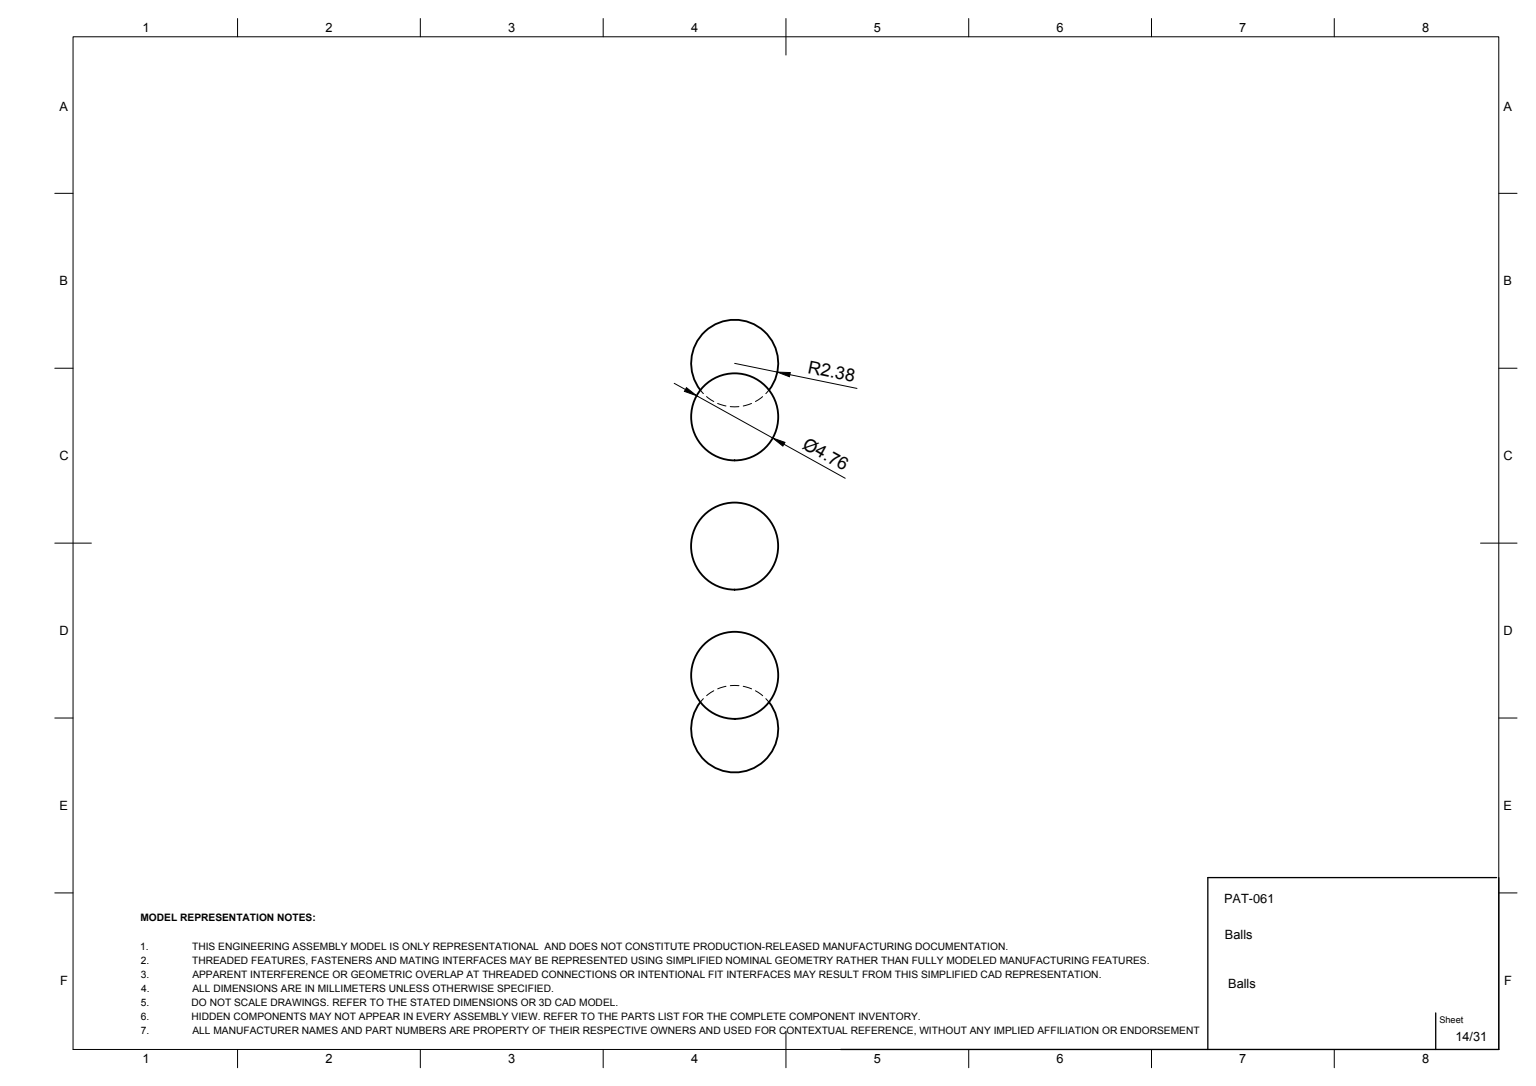
ISO-10303-21;
HEADER;
/* Generated by software containing ST-Developer
 * from STEP Tools, Inc. (www.steptools.com) 
 */

FILE_DESCRIPTION(
/* description */ ('Compact intermittent indexer'),
/* implementation_level */ '2;1');

FILE_NAME(
/* name */ 'Balls.step',
/* time_stamp */ '2026-10-29T16:32:17-07:00',
/* author */ (''),
/* organization */ (''),
/* preprocessor_version */ 'ST-DEVELOPER v20.2',
/* originating_system */ 'Autodesk Translation Framework v15.17.0.0',
/* authorisation */ '');

FILE_SCHEMA (('AUTOMOTIVE_DESIGN { 1 0 10303 214 3 1 1 }'));
ENDSEC;

DATA;
#10=MECHANICAL_DESIGN_GEOMETRIC_PRESENTATION_REPRESENTATION('',(#265,#266,#267,#268,#269,#270,#271,#272),#10837);
#175=SPHERICAL_SURFACE('',#6230,0.23815);
#176=SPHERICAL_SURFACE('',#6232,0.23815);
#177=SPHERICAL_SURFACE('',#6234,0.23815);
#178=SPHERICAL_SURFACE('',#6236,0.23815);
#179=SPHERICAL_SURFACE('',#6238,0.23815);
#180=SPHERICAL_SURFACE('',#6240,0.23815);
#181=SPHERICAL_SURFACE('',#6242,0.23815);
#182=SPHERICAL_SURFACE('',#6244,0.23815);
#217=SHAPE_REPRESENTATION_RELATIONSHIP('SRR','None',#10952,#241);
#241=ADVANCED_BREP_SHAPE_REPRESENTATION('',(#296,#297,#298,#299,#300,#301,
#302,#303),#10819);
#265=STYLED_ITEM('',(#11166),#296);
#266=STYLED_ITEM('',(#11166),#297);
#267=STYLED_ITEM('',(#11166),#298);
#268=STYLED_ITEM('',(#11166),#299);
#269=STYLED_ITEM('',(#11166),#300);
#270=STYLED_ITEM('',(#11166),#301);
#271=STYLED_ITEM('',(#11166),#302);
#272=STYLED_ITEM('',(#11166),#303);
#296=MANIFOLD_SOLID_BREP('Body1',#5638);
#297=MANIFOLD_SOLID_BREP('Body2',#5639);
#298=MANIFOLD_SOLID_BREP('Body3',#5640);
#299=MANIFOLD_SOLID_BREP('Body4',#5641);
#300=MANIFOLD_SOLID_BREP('Body5',#5642);
#301=MANIFOLD_SOLID_BREP('Body6',#5643);
#302=MANIFOLD_SOLID_BREP('Body7',#5644);
#303=MANIFOLD_SOLID_BREP('Body8',#5645);
#794=FACE_OUTER_BOUND('',#1196,.T.);
#795=FACE_OUTER_BOUND('',#1197,.T.);
#796=FACE_OUTER_BOUND('',#1198,.T.);
#797=FACE_OUTER_BOUND('',#1199,.T.);
#798=FACE_OUTER_BOUND('',#1200,.T.);
#799=FACE_OUTER_BOUND('',#1201,.T.);
#800=FACE_OUTER_BOUND('',#1202,.T.);
#801=FACE_OUTER_BOUND('',#1203,.T.);
#1196=EDGE_LOOP('',(#4292,#4293));
#1197=EDGE_LOOP('',(#4294,#4295));
#1198=EDGE_LOOP('',(#4296,#4297));
#1199=EDGE_LOOP('',(#4298,#4299));
#1200=EDGE_LOOP('',(#4300,#4301));
#1201=EDGE_LOOP('',(#4302,#4303));
#1202=EDGE_LOOP('',(#4304,#4305));
#1203=EDGE_LOOP('',(#4306,#4307));
#2296=CIRCLE('',#6231,0.23815);
#2297=CIRCLE('',#6233,0.23815);
#2298=CIRCLE('',#6235,0.23815);
#2299=CIRCLE('',#6237,0.23815);
#2300=CIRCLE('',#6239,0.23815);
#2301=CIRCLE('',#6241,0.23815);
#2302=CIRCLE('',#6243,0.23815);
#2303=CIRCLE('',#6245,0.23815);
#2674=VERTEX_POINT('',#9205);
#2675=VERTEX_POINT('',#9206);
#2676=VERTEX_POINT('',#9209);
#2677=VERTEX_POINT('',#9210);
#2678=VERTEX_POINT('',#9213);
#2679=VERTEX_POINT('',#9214);
#2680=VERTEX_POINT('',#9217);
#2681=VERTEX_POINT('',#9218);
#2682=VERTEX_POINT('',#9221);
#2683=VERTEX_POINT('',#9222);
#2684=VERTEX_POINT('',#9225);
#2685=VERTEX_POINT('',#9226);
#2686=VERTEX_POINT('',#9229);
#2687=VERTEX_POINT('',#9230);
#2688=VERTEX_POINT('',#9233);
#2689=VERTEX_POINT('',#9234);
#3268=EDGE_CURVE('',#2674,#2675,#2296,.T.);
#3269=EDGE_CURVE('',#2676,#2677,#2297,.T.);
#3270=EDGE_CURVE('',#2678,#2679,#2298,.T.);
#3271=EDGE_CURVE('',#2680,#2681,#2299,.T.);
#3272=EDGE_CURVE('',#2682,#2683,#2300,.T.);
#3273=EDGE_CURVE('',#2684,#2685,#2301,.T.);
#3274=EDGE_CURVE('',#2686,#2687,#2302,.T.);
#3275=EDGE_CURVE('',#2688,#2689,#2303,.T.);
#4292=ORIENTED_EDGE('',*,*,#3268,.T.);
#4293=ORIENTED_EDGE('',*,*,#3268,.F.);
#4294=ORIENTED_EDGE('',*,*,#3269,.T.);
#4295=ORIENTED_EDGE('',*,*,#3269,.F.);
#4296=ORIENTED_EDGE('',*,*,#3270,.T.);
#4297=ORIENTED_EDGE('',*,*,#3270,.F.);
#4298=ORIENTED_EDGE('',*,*,#3271,.T.);
#4299=ORIENTED_EDGE('',*,*,#3271,.F.);
#4300=ORIENTED_EDGE('',*,*,#3272,.T.);
#4301=ORIENTED_EDGE('',*,*,#3272,.F.);
#4302=ORIENTED_EDGE('',*,*,#3273,.T.);
#4303=ORIENTED_EDGE('',*,*,#3273,.F.);
#4304=ORIENTED_EDGE('',*,*,#3274,.T.);
#4305=ORIENTED_EDGE('',*,*,#3274,.F.);
#4306=ORIENTED_EDGE('',*,*,#3275,.T.);
#4307=ORIENTED_EDGE('',*,*,#3275,.F.);
#5437=ADVANCED_FACE('',(#794),#175,.T.);
#5438=ADVANCED_FACE('',(#795),#176,.T.);
#5439=ADVANCED_FACE('',(#796),#177,.T.);
#5440=ADVANCED_FACE('',(#797),#178,.T.);
#5441=ADVANCED_FACE('',(#798),#179,.T.);
#5442=ADVANCED_FACE('',(#799),#180,.T.);
#5443=ADVANCED_FACE('',(#800),#181,.T.);
#5444=ADVANCED_FACE('',(#801),#182,.T.);
#5638=CLOSED_SHELL('',(#5437));
#5639=CLOSED_SHELL('',(#5438));
#5640=CLOSED_SHELL('',(#5439));
#5641=CLOSED_SHELL('',(#5440));
#5642=CLOSED_SHELL('',(#5441));
#5643=CLOSED_SHELL('',(#5442));
#5644=CLOSED_SHELL('',(#5443));
#5645=CLOSED_SHELL('',(#5444));
#6229=AXIS2_PLACEMENT_3D('',#9203,#7410,#7411);
#6230=AXIS2_PLACEMENT_3D('',#9204,#7412,#7413);
#6231=AXIS2_PLACEMENT_3D('',#9207,#7414,#7415);
#6232=AXIS2_PLACEMENT_3D('',#9208,#7416,#7417);
#6233=AXIS2_PLACEMENT_3D('',#9211,#7418,#7419);
#6234=AXIS2_PLACEMENT_3D('',#9212,#7420,#7421);
#6235=AXIS2_PLACEMENT_3D('',#9215,#7422,#7423);
#6236=AXIS2_PLACEMENT_3D('',#9216,#7424,#7425);
#6237=AXIS2_PLACEMENT_3D('',#9219,#7426,#7427);
#6238=AXIS2_PLACEMENT_3D('',#9220,#7428,#7429);
#6239=AXIS2_PLACEMENT_3D('',#9223,#7430,#7431);
#6240=AXIS2_PLACEMENT_3D('',#9224,#7432,#7433);
#6241=AXIS2_PLACEMENT_3D('',#9227,#7434,#7435);
#6242=AXIS2_PLACEMENT_3D('',#9228,#7436,#7437);
#6243=AXIS2_PLACEMENT_3D('',#9231,#7438,#7439);
#6244=AXIS2_PLACEMENT_3D('',#9232,#7440,#7441);
#6245=AXIS2_PLACEMENT_3D('',#9235,#7442,#7443);
#7410=DIRECTION('axis',(0.,0.,1.));
#7411=DIRECTION('refdir',(1.,0.,0.));
#7412=DIRECTION('center_axis',(0.,0.,1.));
#7413=DIRECTION('ref_axis',(1.,0.,0.));
#7414=DIRECTION('center_axis',(1.22464679914735E-16,-1.,0.));
#7415=DIRECTION('ref_axis',(-1.,-1.22464679914735E-16,0.));
#7416=DIRECTION('center_axis',(0.707106781186548,0.,0.707106781186548));
#7417=DIRECTION('ref_axis',(0.707106781186548,0.,-0.707106781186548));
#7418=DIRECTION('center_axis',(8.65956056235494E-17,-1.,-8.65956056235493E-17));
#7419=DIRECTION('ref_axis',(-0.707106781186547,-1.22464679914735E-16,0.707106781186547));
#7420=DIRECTION('center_axis',(1.,0.,0.));
#7421=DIRECTION('ref_axis',(6.12323399573676E-17,0.,-1.));
#7422=DIRECTION('center_axis',(7.49879891330929E-33,-1.,-1.22464679914735E-16));
#7423=DIRECTION('ref_axis',(-6.12323399573676E-17,-1.22464679914735E-16,
1.));
#7424=DIRECTION('center_axis',(0.707106781186548,0.,-0.707106781186548));
#7425=DIRECTION('ref_axis',(-0.707106781186548,0.,-0.707106781186548));
#7426=DIRECTION('center_axis',(-8.65956056235493E-17,-1.,-8.65956056235494E-17));
#7427=DIRECTION('ref_axis',(0.707106781186547,-1.22464679914735E-16,0.707106781186547));
#7428=DIRECTION('center_axis',(0.,0.,-1.));
#7429=DIRECTION('ref_axis',(-1.,0.,-1.22464679914735E-16));
#7430=DIRECTION('center_axis',(-1.22464679914735E-16,-1.,-1.49975978266186E-32));
#7431=DIRECTION('ref_axis',(1.,-1.22464679914735E-16,1.22464679914735E-16));
#7432=DIRECTION('center_axis',(-0.707106781186547,0.,-0.707106781186548));
#7433=DIRECTION('ref_axis',(-0.707106781186548,0.,0.707106781186547));
#7434=DIRECTION('center_axis',(-8.65956056235493E-17,-1.,8.65956056235493E-17));
#7435=DIRECTION('ref_axis',(0.707106781186548,-1.22464679914735E-16,-0.707106781186547));
#7436=DIRECTION('center_axis',(-1.,0.,0.));
#7437=DIRECTION('ref_axis',(-1.83697019872103E-16,0.,1.));
#7438=DIRECTION('center_axis',(-2.24963967399279E-32,-1.,1.22464679914735E-16));
#7439=DIRECTION('ref_axis',(1.83697019872103E-16,-1.22464679914735E-16,
-1.));
#7440=DIRECTION('center_axis',(-0.707106781186548,0.,0.707106781186548));
#7441=DIRECTION('ref_axis',(0.707106781186547,0.,0.707106781186548));
#7442=DIRECTION('center_axis',(8.65956056235493E-17,-1.,8.65956056235493E-17));
#7443=DIRECTION('ref_axis',(-0.707106781186547,-1.22464679914735E-16,-0.707106781186548));
#9203=CARTESIAN_POINT('',(0.,0.,0.));
#9204=CARTESIAN_POINT('Origin',(1.,0.,0.));
#9205=CARTESIAN_POINT('',(1.,-1.78583896120461E-33,0.23815));
#9206=CARTESIAN_POINT('',(1.,-1.78583896120461E-33,-0.23815));
#9207=CARTESIAN_POINT('Origin',(1.,0.,0.));
#9208=CARTESIAN_POINT('Origin',(0.707106781186548,0.,-0.707106781186547));
#9209=CARTESIAN_POINT('',(0.875504261126124,-1.78583896120461E-33,-0.538709301246971));
#9210=CARTESIAN_POINT('',(0.538709301246971,-1.78583896120461E-33,-0.875504261126124));
#9211=CARTESIAN_POINT('Origin',(0.707106781186548,0.,-0.707106781186547));
#9212=CARTESIAN_POINT('Origin',(6.12323399573677E-17,0.,-1.));
#9213=CARTESIAN_POINT('',(0.23815,-1.78583896120461E-33,-1.));
#9214=CARTESIAN_POINT('',(-0.23815,-1.78583896120461E-33,-1.));
#9215=CARTESIAN_POINT('Origin',(6.12323399573677E-17,0.,-1.));
#9216=CARTESIAN_POINT('Origin',(-0.707106781186547,0.,-0.707106781186548));
#9217=CARTESIAN_POINT('',(-0.538709301246971,-1.78583896120461E-33,-0.875504261126124));
#9218=CARTESIAN_POINT('',(-0.875504261126124,-1.78583896120461E-33,-0.538709301246971));
#9219=CARTESIAN_POINT('Origin',(-0.707106781186547,0.,-0.707106781186548));
#9220=CARTESIAN_POINT('Origin',(-1.,0.,-1.22464679914735E-16));
#9221=CARTESIAN_POINT('',(-1.,-1.78583896120461E-33,-0.23815));
#9222=CARTESIAN_POINT('',(-1.,-1.78583896120461E-33,0.23815));
#9223=CARTESIAN_POINT('Origin',(-1.,0.,-1.22464679914735E-16));
#9224=CARTESIAN_POINT('Origin',(-0.707106781186548,0.,0.707106781186547));
#9225=CARTESIAN_POINT('',(-0.875504261126124,-7.94881478324376E-33,0.538709301246971));
#9226=CARTESIAN_POINT('',(-0.538709301246971,4.37713686083455E-33,0.875504261126124));
#9227=CARTESIAN_POINT('Origin',(-0.707106781186548,0.,0.707106781186547));
#9228=CARTESIAN_POINT('Origin',(-1.83697019872103E-16,0.,1.));
#9229=CARTESIAN_POINT('',(-0.23815,-1.78583896120461E-33,1.));
#9230=CARTESIAN_POINT('',(0.23815,-1.78583896120461E-33,1.));
#9231=CARTESIAN_POINT('Origin',(-1.83697019872103E-16,0.,1.));
#9232=CARTESIAN_POINT('Origin',(0.707106781186547,0.,0.707106781186548));
#9233=CARTESIAN_POINT('',(0.538709301246971,-4.86732687222419E-33,0.875504261126124));
#9234=CARTESIAN_POINT('',(0.875504261126124,1.29564894981497E-33,0.538709301246971));
#9235=CARTESIAN_POINT('Origin',(0.707106781186547,0.,0.707106781186548));
#10789=UNCERTAINTY_MEASURE_WITH_UNIT(LENGTH_MEASURE(0.001),#10838,
'DISTANCE_ACCURACY_VALUE',
'Maximum model space distance between geometric entities at asserted c
onnectivities');
#10807=UNCERTAINTY_MEASURE_WITH_UNIT(LENGTH_MEASURE(0.001),#10838,
'DISTANCE_ACCURACY_VALUE',
'Maximum model space distance between geometric entities at asserted c
onnectivities');
#10819=(
GEOMETRIC_REPRESENTATION_CONTEXT(3)
GLOBAL_UNCERTAINTY_ASSIGNED_CONTEXT((#10789))
GLOBAL_UNIT_ASSIGNED_CONTEXT((#10838,#10840,#10841))
REPRESENTATION_CONTEXT('','3D')
);
#10837=(
GEOMETRIC_REPRESENTATION_CONTEXT(3)
GLOBAL_UNCERTAINTY_ASSIGNED_CONTEXT((#10807))
GLOBAL_UNIT_ASSIGNED_CONTEXT((#10838,#10840,#10841))
REPRESENTATION_CONTEXT('','3D')
);
#10838=(
LENGTH_UNIT()
NAMED_UNIT(*)
SI_UNIT(.CENTI.,.METRE.)
);
#10840=(
NAMED_UNIT(*)
PLANE_ANGLE_UNIT()
SI_UNIT($,.RADIAN.)
);
#10841=(
NAMED_UNIT(*)
SI_UNIT($,.STERADIAN.)
SOLID_ANGLE_UNIT()
);
#10853=SHAPE_DEFINITION_REPRESENTATION(#10882,#10952);
#10882=PRODUCT_DEFINITION_SHAPE('',$,#10982);
#10952=SHAPE_REPRESENTATION('',(#6229),#10819);
#10970=PRODUCT_DEFINITION_CONTEXT('part definition',#11059,'design');
#10982=PRODUCT_DEFINITION('Balls','Balls',#11011,#10970);
#11011=PRODUCT_DEFINITION_FORMATION('',$,#11072);
#11059=APPLICATION_CONTEXT(
'Core Data for Automotive Mechanical Design Process');
#11060=PRODUCT_CONTEXT('part definition',#11059,'mechanical');
#11072=PRODUCT('Balls','Balls','Balls',(#11060));
#11160=COLOUR_RGB('Grey',0.48,0.52,0.57);
#11161=FILL_AREA_STYLE_COLOUR('',#11160);
#11162=FILL_AREA_STYLE('',(#11161));
#11163=SURFACE_STYLE_FILL_AREA(#11162);
#11164=SURFACE_SIDE_STYLE('',(#11163));
#11165=SURFACE_STYLE_USAGE(.BOTH.,#11164);
#11166=PRESENTATION_STYLE_ASSIGNMENT((#11165));
ENDSEC;
END-ISO-10303-21;
